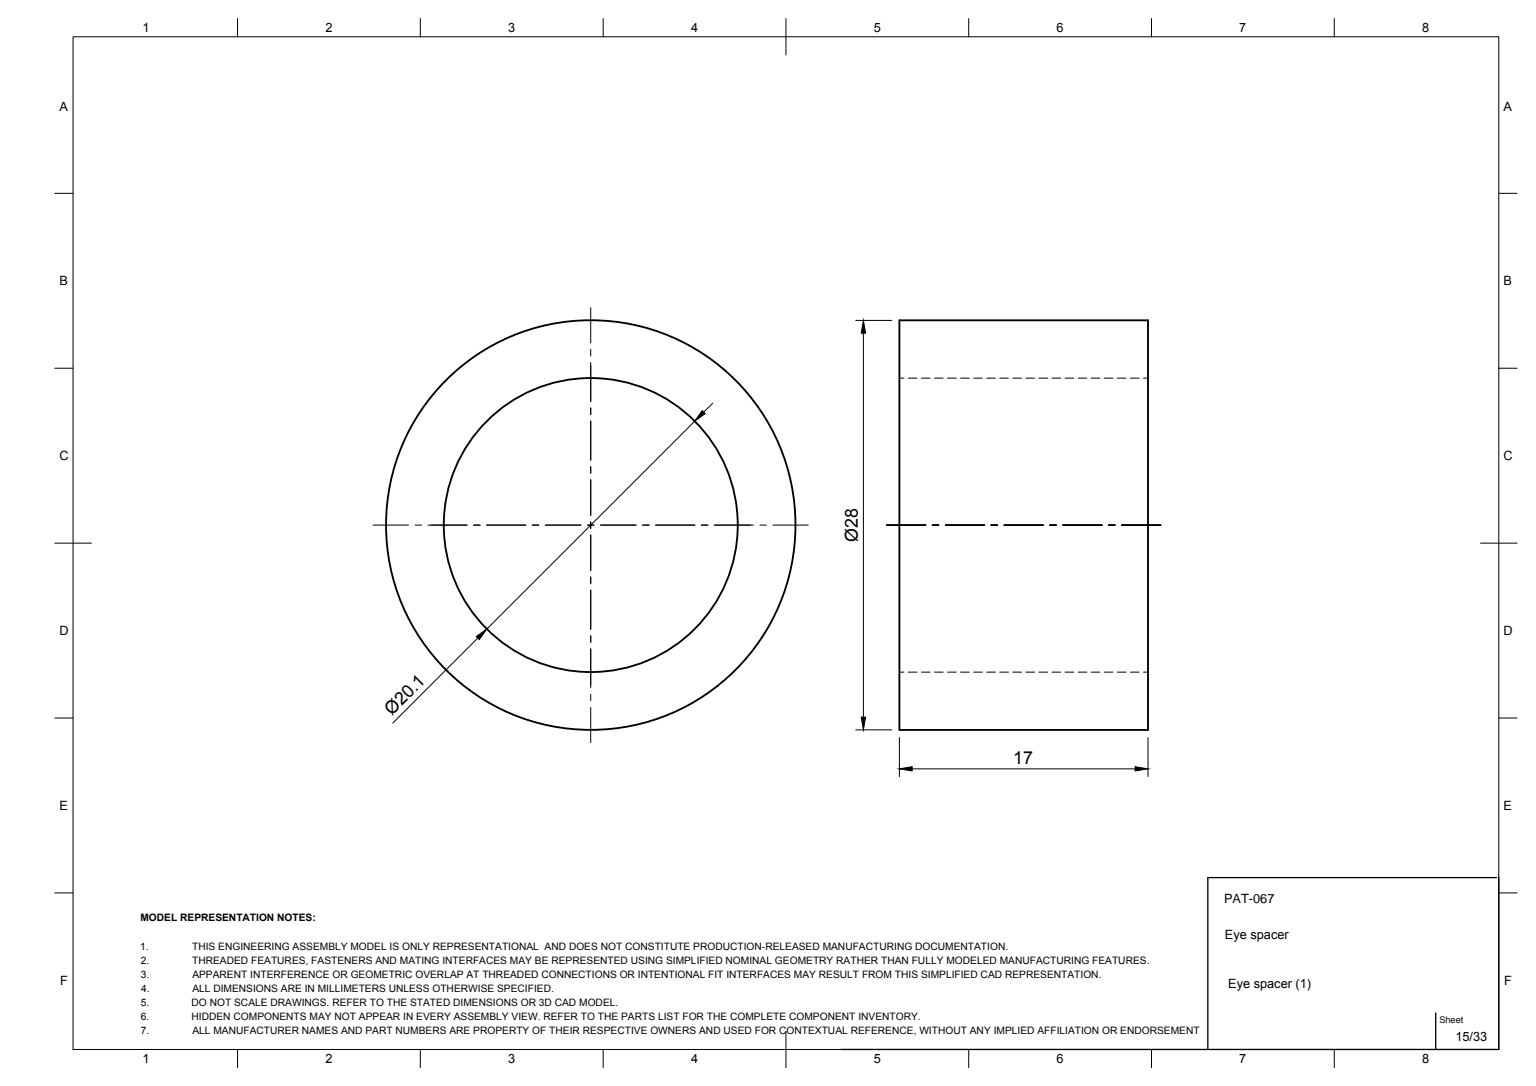
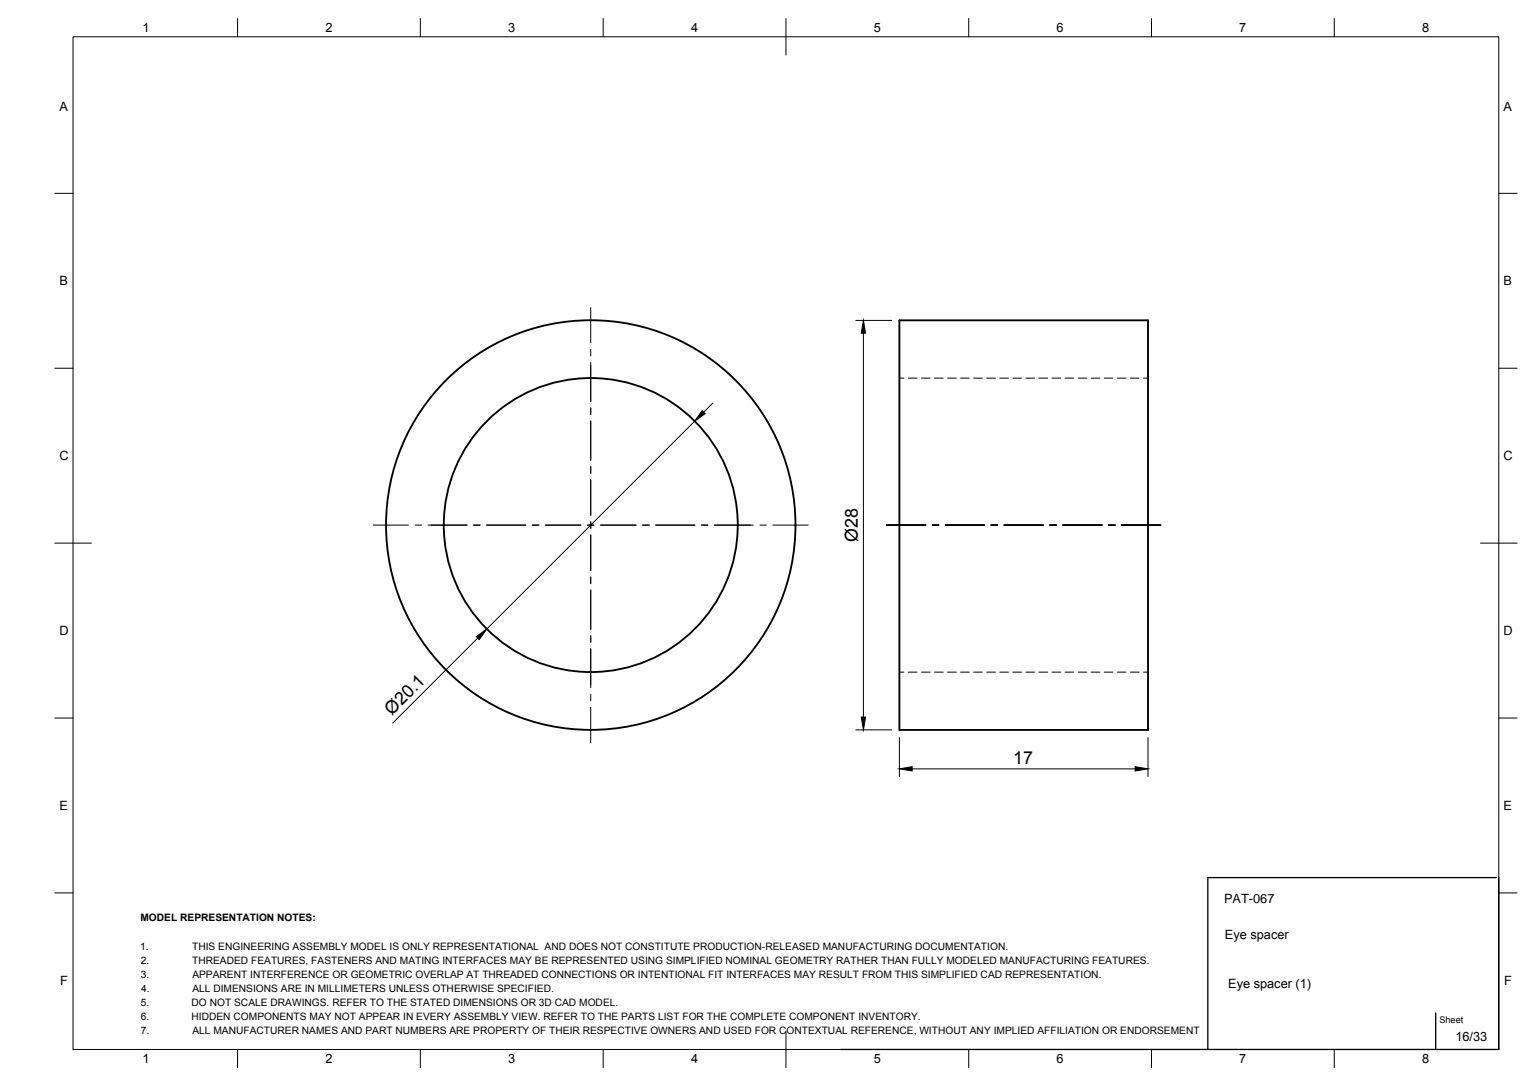
ISO-10303-21;
HEADER;
/* Generated by software containing ST-Developer
 * from STEP Tools, Inc. (www.steptools.com) 
 */

FILE_DESCRIPTION(
/* description */ ('Lifting hook block with sheave'),
/* implementation_level */ '2;1');

FILE_NAME(
/* name */ 'Eye spacer.step',
/* time_stamp */ '2026-10-28T03:23:54-07:00',
/* author */ (''),
/* organization */ (''),
/* preprocessor_version */ 'ST-DEVELOPER v20.2',
/* originating_system */ 'Autodesk Translation Framework v15.17.0.0',
/* authorisation */ '');

FILE_SCHEMA (('AUTOMOTIVE_DESIGN { 1 0 10303 214 3 1 1 }'));
ENDSEC;

DATA;
#10=MECHANICAL_DESIGN_GEOMETRIC_PRESENTATION_REPRESENTATION('',(#361),#9391);
#301=SHAPE_REPRESENTATION_RELATIONSHIP('SRR','None',#9532,#331);
#331=ADVANCED_BREP_SHAPE_REPRESENTATION('',(#399),#9367);
#361=STYLED_ITEM('',(#9745),#399);
#399=MANIFOLD_SOLID_BREP('Body1',#4897);
#536=LINE('',#8024,#824);
#537=LINE('',#8030,#825);
#824=VECTOR('',#6459,1.005);
#825=VECTOR('',#6466,1.4);
#1044=CYLINDRICAL_SURFACE('',#5466,1.005);
#1045=CYLINDRICAL_SURFACE('',#5469,1.4);
#1155=FACE_BOUND('',#1652,.T.);
#1156=FACE_BOUND('',#1654,.T.);
#1312=FACE_OUTER_BOUND('',#1649,.T.);
#1313=FACE_OUTER_BOUND('',#1650,.T.);
#1314=FACE_OUTER_BOUND('',#1651,.T.);
#1315=FACE_OUTER_BOUND('',#1653,.T.);
#1649=EDGE_LOOP('',(#3662,#3663,#3664,#3665));
#1650=EDGE_LOOP('',(#3666,#3667,#3668,#3669));
#1651=EDGE_LOOP('',(#3670));
#1652=EDGE_LOOP('',(#3671));
#1653=EDGE_LOOP('',(#3672));
#1654=EDGE_LOOP('',(#3673));
#2019=CIRCLE('',#5467,1.005);
#2020=CIRCLE('',#5468,1.005);
#2021=CIRCLE('',#5470,1.4);
#2022=CIRCLE('',#5471,1.4);
#2352=VERTEX_POINT('',#8021);
#2353=VERTEX_POINT('',#8023);
#2354=VERTEX_POINT('',#8027);
#2355=VERTEX_POINT('',#8029);
#2835=EDGE_CURVE('',#2352,#2352,#2019,.T.);
#2836=EDGE_CURVE('',#2352,#2353,#536,.T.);
#2837=EDGE_CURVE('',#2353,#2353,#2020,.T.);
#2838=EDGE_CURVE('',#2354,#2354,#2021,.T.);
#2839=EDGE_CURVE('',#2354,#2355,#537,.T.);
#2840=EDGE_CURVE('',#2355,#2355,#2022,.T.);
#3662=ORIENTED_EDGE('',*,*,#2835,.F.);
#3663=ORIENTED_EDGE('',*,*,#2836,.T.);
#3664=ORIENTED_EDGE('',*,*,#2837,.T.);
#3665=ORIENTED_EDGE('',*,*,#2836,.F.);
#3666=ORIENTED_EDGE('',*,*,#2838,.F.);
#3667=ORIENTED_EDGE('',*,*,#2839,.T.);
#3668=ORIENTED_EDGE('',*,*,#2840,.T.);
#3669=ORIENTED_EDGE('',*,*,#2839,.F.);
#3670=ORIENTED_EDGE('',*,*,#2838,.T.);
#3671=ORIENTED_EDGE('',*,*,#2835,.T.);
#3672=ORIENTED_EDGE('',*,*,#2840,.F.);
#3673=ORIENTED_EDGE('',*,*,#2837,.F.);
#4498=PLANE('',#5472);
#4499=PLANE('',#5473);
#4688=ADVANCED_FACE('',(#1312),#1044,.F.);
#4689=ADVANCED_FACE('',(#1313),#1045,.T.);
#4690=ADVANCED_FACE('',(#1314,#1155),#4498,.T.);
#4691=ADVANCED_FACE('',(#1315,#1156),#4499,.F.);
#4897=CLOSED_SHELL('',(#4688,#4689,#4690,#4691));
#5465=AXIS2_PLACEMENT_3D('',#8019,#6453,#6454);
#5466=AXIS2_PLACEMENT_3D('',#8020,#6455,#6456);
#5467=AXIS2_PLACEMENT_3D('',#8022,#6457,#6458);
#5468=AXIS2_PLACEMENT_3D('',#8025,#6460,#6461);
#5469=AXIS2_PLACEMENT_3D('',#8026,#6462,#6463);
#5470=AXIS2_PLACEMENT_3D('',#8028,#6464,#6465);
#5471=AXIS2_PLACEMENT_3D('',#8031,#6467,#6468);
#5472=AXIS2_PLACEMENT_3D('',#8032,#6469,#6470);
#5473=AXIS2_PLACEMENT_3D('',#8033,#6471,#6472);
#6453=DIRECTION('axis',(0.,0.,1.));
#6454=DIRECTION('refdir',(1.,0.,0.));
#6455=DIRECTION('center_axis',(0.,1.,0.));
#6456=DIRECTION('ref_axis',(1.,0.,0.));
#6457=DIRECTION('center_axis',(0.,-1.,0.));
#6458=DIRECTION('ref_axis',(1.,0.,0.));
#6459=DIRECTION('',(0.,-1.,0.));
#6460=DIRECTION('center_axis',(0.,-1.,0.));
#6461=DIRECTION('ref_axis',(1.,0.,0.));
#6462=DIRECTION('center_axis',(0.,1.,0.));
#6463=DIRECTION('ref_axis',(1.,0.,0.));
#6464=DIRECTION('center_axis',(0.,1.,0.));
#6465=DIRECTION('ref_axis',(1.,0.,0.));
#6466=DIRECTION('',(0.,-1.,0.));
#6467=DIRECTION('center_axis',(0.,1.,0.));
#6468=DIRECTION('ref_axis',(1.,0.,0.));
#6469=DIRECTION('center_axis',(0.,1.,0.));
#6470=DIRECTION('ref_axis',(1.,0.,0.));
#6471=DIRECTION('center_axis',(0.,1.,0.));
#6472=DIRECTION('ref_axis',(1.,0.,0.));
#8019=CARTESIAN_POINT('',(0.,0.,0.));
#8020=CARTESIAN_POINT('Origin',(0.,-2.5,20.5));
#8021=CARTESIAN_POINT('',(-1.005,-0.8,20.5));
#8022=CARTESIAN_POINT('Origin',(0.,-0.8,20.5));
#8023=CARTESIAN_POINT('',(-1.005,-2.5,20.5));
#8024=CARTESIAN_POINT('',(-1.005,-2.5,20.5));
#8025=CARTESIAN_POINT('Origin',(0.,-2.5,20.5));
#8026=CARTESIAN_POINT('Origin',(0.,-2.5,20.5));
#8027=CARTESIAN_POINT('',(-1.4,-0.8,20.5));
#8028=CARTESIAN_POINT('Origin',(0.,-0.8,20.5));
#8029=CARTESIAN_POINT('',(-1.4,-2.5,20.5));
#8030=CARTESIAN_POINT('',(-1.4,-2.5,20.5));
#8031=CARTESIAN_POINT('Origin',(0.,-2.5,20.5));
#8032=CARTESIAN_POINT('Origin',(0.,-0.8,20.5));
#8033=CARTESIAN_POINT('Origin',(0.,-2.5,20.5));
#9330=UNCERTAINTY_MEASURE_WITH_UNIT(LENGTH_MEASURE(0.001),#9392,
'DISTANCE_ACCURACY_VALUE',
'Maximum model space distance between geometric entities at asserted c
onnectivities');
#9354=UNCERTAINTY_MEASURE_WITH_UNIT(LENGTH_MEASURE(0.001),#9392,
'DISTANCE_ACCURACY_VALUE',
'Maximum model space distance between geometric entities at asserted c
onnectivities');
#9367=(
GEOMETRIC_REPRESENTATION_CONTEXT(3)
GLOBAL_UNCERTAINTY_ASSIGNED_CONTEXT((#9330))
GLOBAL_UNIT_ASSIGNED_CONTEXT((#9392,#9394,#9395))
REPRESENTATION_CONTEXT('','3D')
);
#9391=(
GEOMETRIC_REPRESENTATION_CONTEXT(3)
GLOBAL_UNCERTAINTY_ASSIGNED_CONTEXT((#9354))
GLOBAL_UNIT_ASSIGNED_CONTEXT((#9392,#9394,#9395))
REPRESENTATION_CONTEXT('','3D')
);
#9392=(
LENGTH_UNIT()
NAMED_UNIT(*)
SI_UNIT(.CENTI.,.METRE.)
);
#9394=(
NAMED_UNIT(*)
PLANE_ANGLE_UNIT()
SI_UNIT($,.RADIAN.)
);
#9395=(
NAMED_UNIT(*)
SI_UNIT($,.STERADIAN.)
SOLID_ANGLE_UNIT()
);
#9408=SHAPE_DEFINITION_REPRESENTATION(#9444,#9532);
#9444=PRODUCT_DEFINITION_SHAPE('',$,#9569);
#9532=SHAPE_REPRESENTATION('',(#5465),#9367);
#9556=PRODUCT_DEFINITION_CONTEXT('part definition',#9666,'design');
#9569=PRODUCT_DEFINITION('Eye spacer','Eye spacer',#9605,#9556);
#9605=PRODUCT_DEFINITION_FORMATION('',$,#9680);
#9666=APPLICATION_CONTEXT(
'Core Data for Automotive Mechanical Design Process');
#9667=PRODUCT_CONTEXT('part definition',#9666,'mechanical');
#9680=PRODUCT('Eye spacer','Eye spacer','Eye spacer',(#9667));
#9739=COLOUR_RGB('Light Blue',0.38,0.62,0.78);
#9740=FILL_AREA_STYLE_COLOUR('',#9739);
#9741=FILL_AREA_STYLE('',(#9740));
#9742=SURFACE_STYLE_FILL_AREA(#9741);
#9743=SURFACE_SIDE_STYLE('',(#9742));
#9744=SURFACE_STYLE_USAGE(.BOTH.,#9743);
#9745=PRESENTATION_STYLE_ASSIGNMENT((#9744));
ENDSEC;
END-ISO-10303-21;
